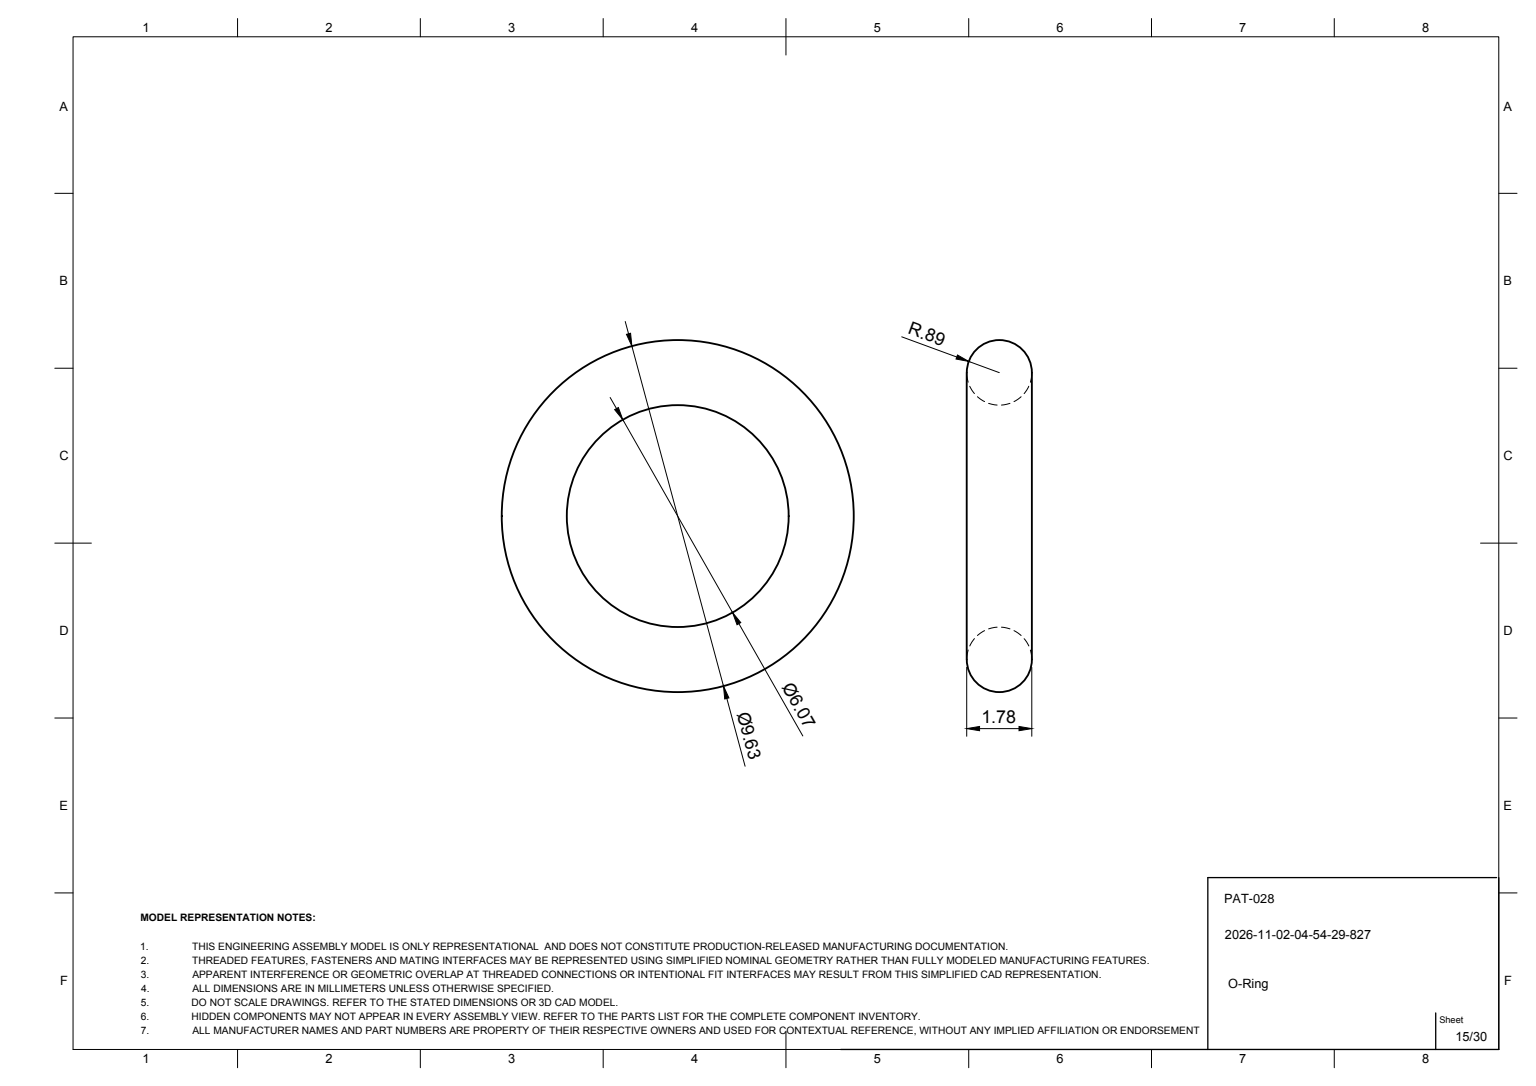
ISO-10303-21;
HEADER;
/* Generated by software containing ST-Developer
 * from STEP Tools, Inc. (www.steptools.com) 
 */

FILE_DESCRIPTION(
/* description */ ('Cylinder foot and clevis mount kit'),
/* implementation_level */ '2;1');

FILE_NAME(
/* name */ 'O-Ring.step',
/* time_stamp */ '2026-10-27T20:10:43-07:00',
/* author */ (''),
/* organization */ (''),
/* preprocessor_version */ 'ST-DEVELOPER v20.2',
/* originating_system */ 'Autodesk Translation Framework v15.17.0.0',
/* authorisation */ '');

FILE_SCHEMA (('AUTOMOTIVE_DESIGN { 1 0 10303 214 3 1 1 }'));
ENDSEC;

DATA;
#10=MECHANICAL_DESIGN_GEOMETRIC_PRESENTATION_REPRESENTATION('',(#351),#9102);
#31=TOROIDAL_SURFACE('',#5639,0.3925,0.089);
#295=SHAPE_REPRESENTATION_RELATIONSHIP('SRR','None',#9243,#323);
#323=ADVANCED_BREP_SHAPE_REPRESENTATION('',(#378),#9086);
#351=STYLED_ITEM('',(#9467),#378);
#378=MANIFOLD_SOLID_BREP('Body1',#4938);
#894=FACE_OUTER_BOUND('',#1274,.T.);
#1274=EDGE_LOOP('',(#4105,#4106,#4107,#4108));
#2252=CIRCLE('',#5640,0.089);
#2253=CIRCLE('',#5641,0.3035);
#2578=VERTEX_POINT('',#8360);
#3107=EDGE_CURVE('',#2578,#2578,#2252,.T.);
#3108=EDGE_CURVE('',#2578,#2578,#2253,.T.);
#4105=ORIENTED_EDGE('',*,*,#3107,.F.);
#4106=ORIENTED_EDGE('',*,*,#3108,.T.);
#4107=ORIENTED_EDGE('',*,*,#3107,.T.);
#4108=ORIENTED_EDGE('',*,*,#3108,.F.);
#4817=ADVANCED_FACE('',(#894),#31,.T.);
#4938=CLOSED_SHELL('',(#4817));
#5638=AXIS2_PLACEMENT_3D('',#8358,#6878,#6879);
#5639=AXIS2_PLACEMENT_3D('',#8359,#6880,#6881);
#5640=AXIS2_PLACEMENT_3D('',#8361,#6882,#6883);
#5641=AXIS2_PLACEMENT_3D('',#8362,#6884,#6885);
#6878=DIRECTION('axis',(0.,0.,1.));
#6879=DIRECTION('refdir',(1.,0.,0.));
#6880=DIRECTION('center_axis',(0.,-1.,0.));
#6881=DIRECTION('ref_axis',(0.,0.,-1.));
#6882=DIRECTION('center_axis',(-1.,0.,-1.22464679914735E-16));
#6883=DIRECTION('ref_axis',(-1.22464679914735E-16,0.,1.));
#6884=DIRECTION('center_axis',(0.,1.,0.));
#6885=DIRECTION('ref_axis',(0.,0.,-1.));
#8358=CARTESIAN_POINT('',(0.,0.,0.));
#8359=CARTESIAN_POINT('Origin',(0.,0.,0.));
#8360=CARTESIAN_POINT('',(-3.71680303541222E-17,-1.08993565124114E-17,0.3035));
#8361=CARTESIAN_POINT('Origin',(-4.80673868665336E-17,0.,0.3925));
#8362=CARTESIAN_POINT('Origin',(0.,1.08993565124114E-17,0.));
#9053=UNCERTAINTY_MEASURE_WITH_UNIT(LENGTH_MEASURE(0.001),#9103,
'DISTANCE_ACCURACY_VALUE',
'Maximum model space distance between geometric entities at asserted c
onnectivities');
#9069=UNCERTAINTY_MEASURE_WITH_UNIT(LENGTH_MEASURE(0.001),#9103,
'DISTANCE_ACCURACY_VALUE',
'Maximum model space distance between geometric entities at asserted c
onnectivities');
#9086=(
GEOMETRIC_REPRESENTATION_CONTEXT(3)
GLOBAL_UNCERTAINTY_ASSIGNED_CONTEXT((#9053))
GLOBAL_UNIT_ASSIGNED_CONTEXT((#9103,#9105,#9106))
REPRESENTATION_CONTEXT('','3D')
);
#9102=(
GEOMETRIC_REPRESENTATION_CONTEXT(3)
GLOBAL_UNCERTAINTY_ASSIGNED_CONTEXT((#9069))
GLOBAL_UNIT_ASSIGNED_CONTEXT((#9103,#9105,#9106))
REPRESENTATION_CONTEXT('','3D')
);
#9103=(
LENGTH_UNIT()
NAMED_UNIT(*)
SI_UNIT(.CENTI.,.METRE.)
);
#9105=(
NAMED_UNIT(*)
PLANE_ANGLE_UNIT()
SI_UNIT($,.RADIAN.)
);
#9106=(
NAMED_UNIT(*)
SI_UNIT($,.STERADIAN.)
SOLID_ANGLE_UNIT()
);
#9123=SHAPE_DEFINITION_REPRESENTATION(#9157,#9243);
#9157=PRODUCT_DEFINITION_SHAPE('',$,#9276);
#9243=SHAPE_REPRESENTATION('',(#5638),#9086);
#9259=PRODUCT_DEFINITION_CONTEXT('part definition',#9357,'design');
#9276=PRODUCT_DEFINITION('O-Ring','O-Ring',#9308,#9259);
#9308=PRODUCT_DEFINITION_FORMATION('',$,#9375);
#9357=APPLICATION_CONTEXT(
'Core Data for Automotive Mechanical Design Process');
#9358=PRODUCT_CONTEXT('part definition',#9357,'mechanical');
#9375=PRODUCT('O-Ring','O-Ring','O-Ring',(#9358));
#9461=COLOUR_RGB('Black',0.12,0.14,0.17);
#9462=FILL_AREA_STYLE_COLOUR('',#9461);
#9463=FILL_AREA_STYLE('',(#9462));
#9464=SURFACE_STYLE_FILL_AREA(#9463);
#9465=SURFACE_SIDE_STYLE('',(#9464));
#9466=SURFACE_STYLE_USAGE(.BOTH.,#9465);
#9467=PRESENTATION_STYLE_ASSIGNMENT((#9466));
ENDSEC;
END-ISO-10303-21;
